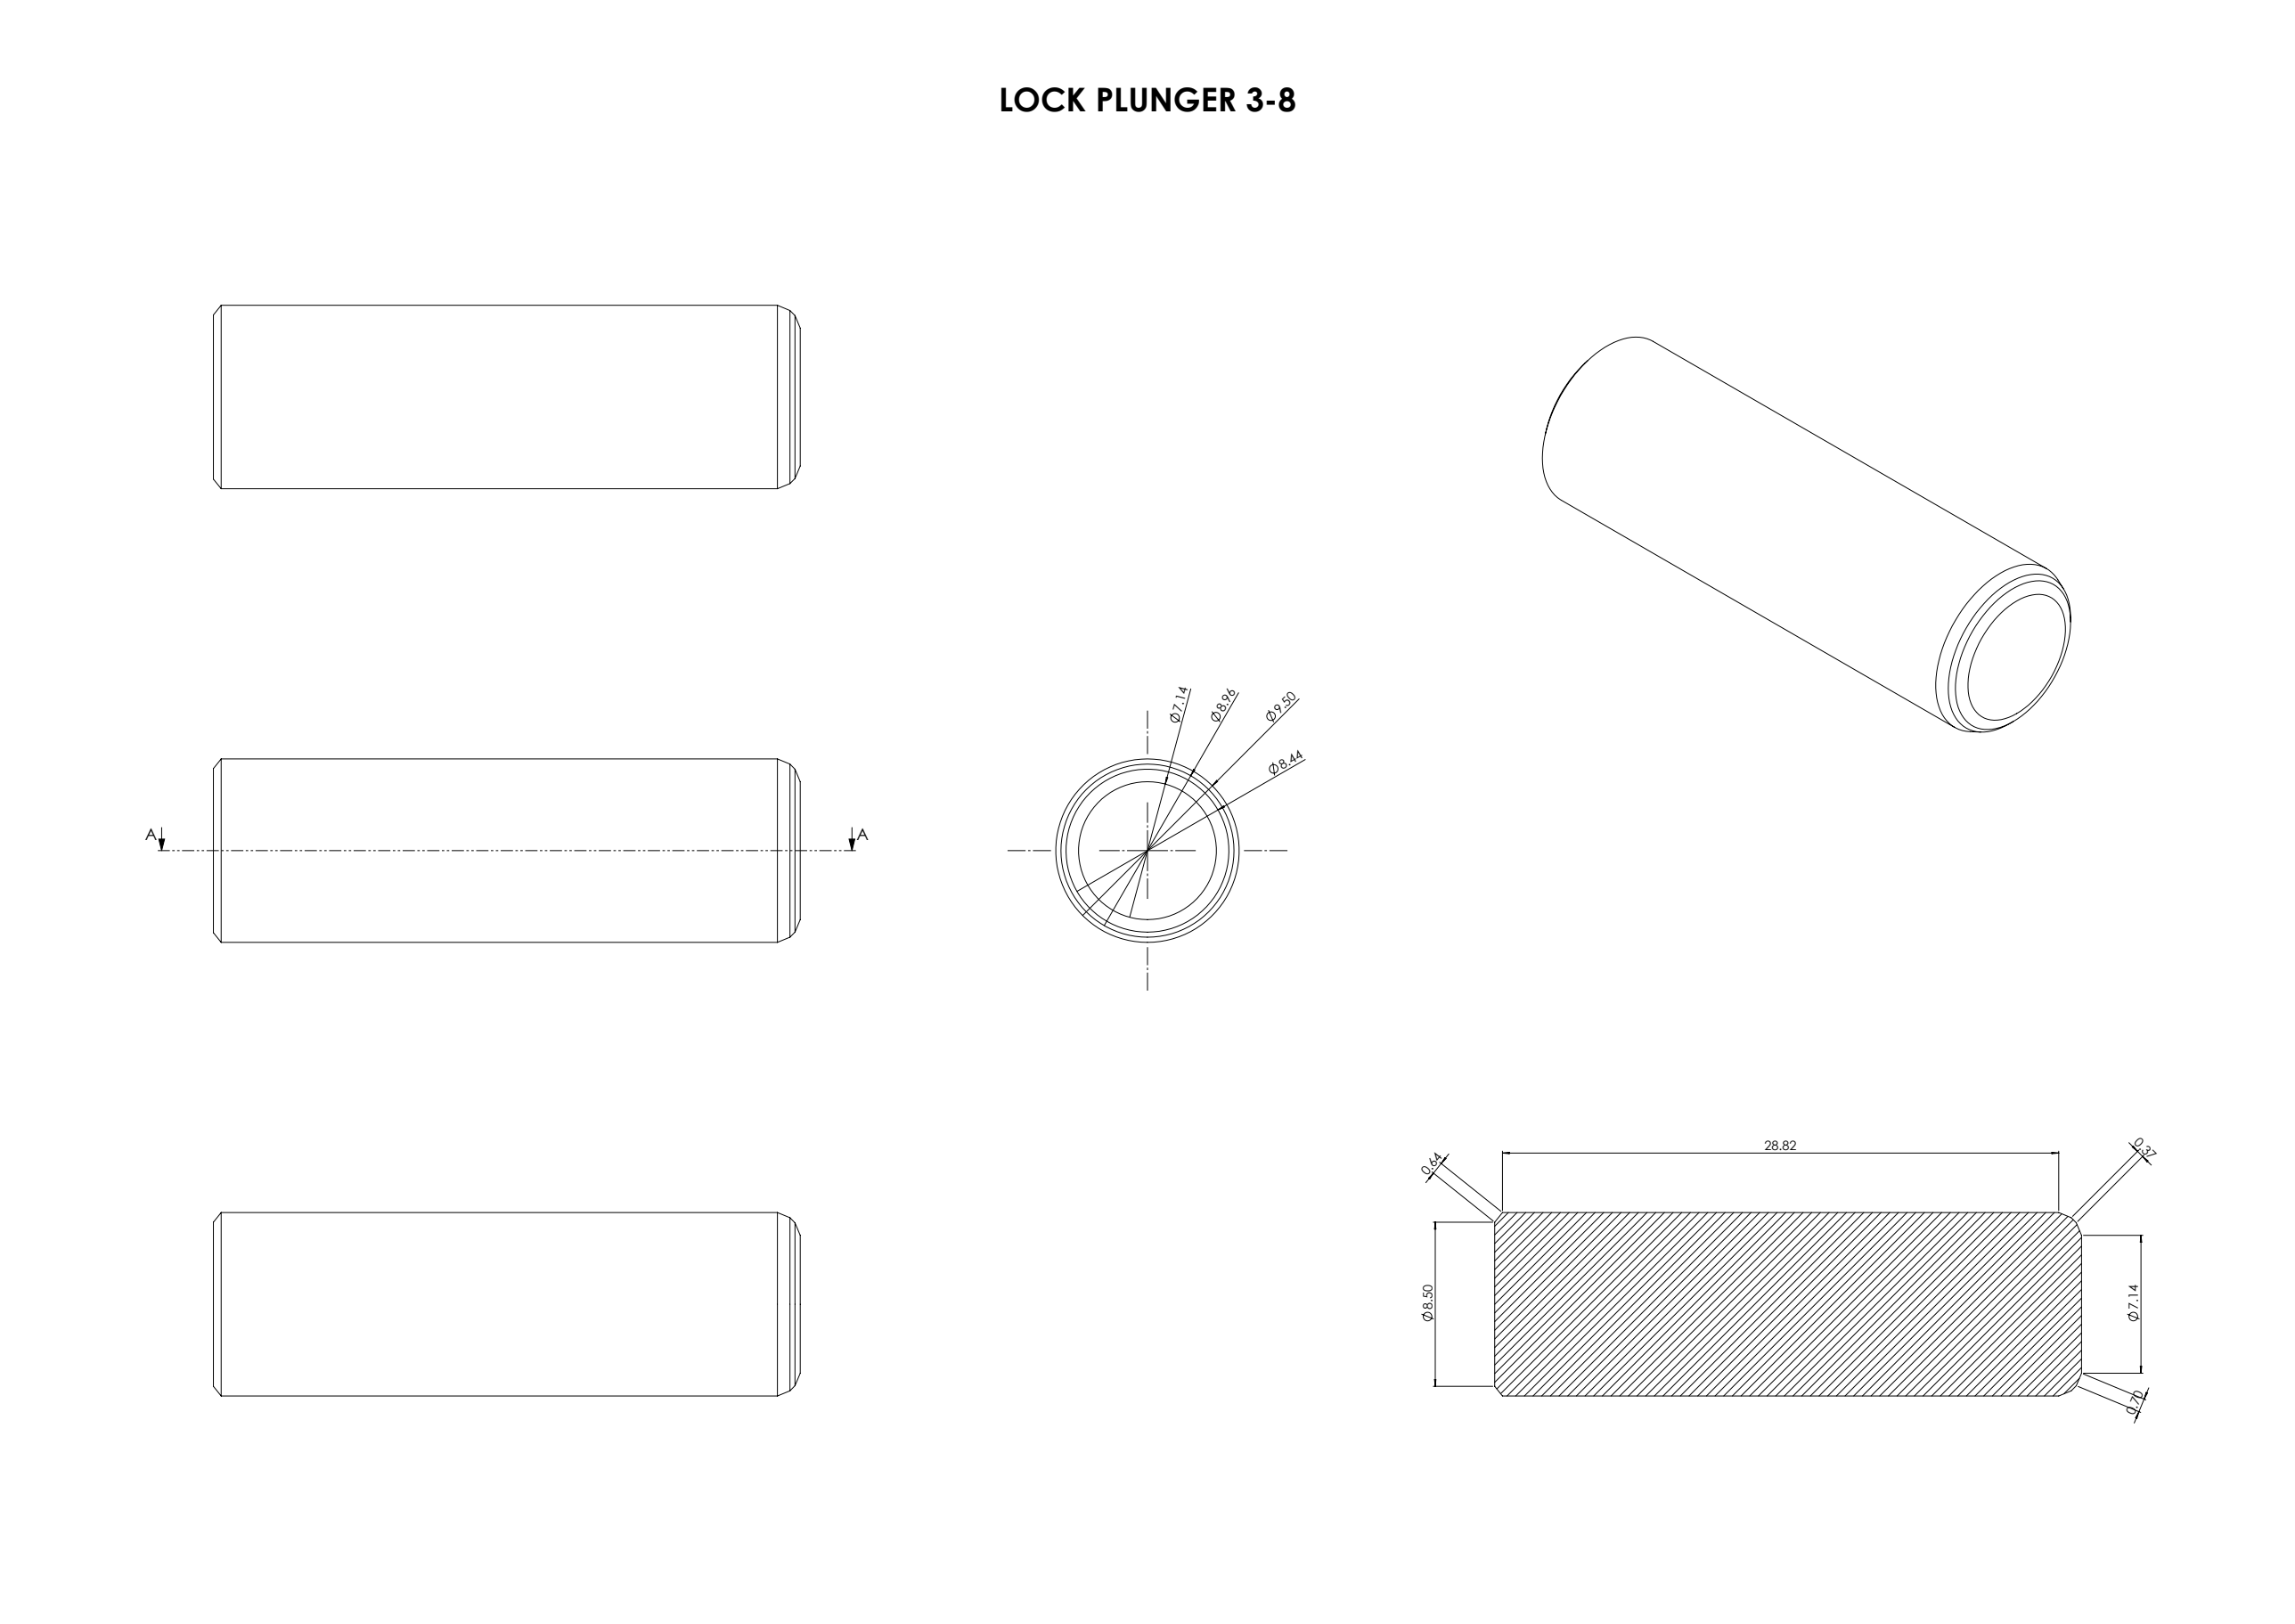
ISO-10303-21;
HEADER;
/* Generated by software containing ST-Developer
 * from STEP Tools, Inc. (www.steptools.com) 
 */

FILE_DESCRIPTION(
/* description */ (''),
/* implementation_level */ '2;1');

FILE_NAME(
/* name */ '09_Lock_Plunger_3-8.step',
/* time_stamp */ '2026-10-25T01:30:15-07:00',
/* author */ (''),
/* organization */ (''),
/* preprocessor_version */ 'ST-DEVELOPER v20.2',
/* originating_system */ 'Autodesk Translation Framework v15.15.0.0',
/* authorisation */ '');

FILE_SCHEMA (('AUTOMOTIVE_DESIGN { 1 0 10303 214 3 1 1 }'));
ENDSEC;

DATA;
#10=MECHANICAL_DESIGN_GEOMETRIC_PRESENTATION_REPRESENTATION('',(#571),#32309);
#543=SHAPE_REPRESENTATION_RELATIONSHIP('SRR','None',#32370,#557);
#557=ADVANCED_BREP_SHAPE_REPRESENTATION('',(#585),#32303);
#571=STYLED_ITEM('',(#32495),#585);
#585=MANIFOLD_SOLID_BREP('Body1',#13812);
#742=CYLINDRICAL_SURFACE('',#14622,4.75);
#1008=CIRCLE('',#14612,3.57);
#1009=CIRCLE('',#14613,4.21870057685089);
#1010=CIRCLE('',#14614,4.21870057685089);
#1011=CIRCLE('',#14616,4.48129942314911);
#1012=CIRCLE('',#14617,4.48129942314911);
#1013=CIRCLE('',#14620,4.75);
#1014=CIRCLE('',#14621,4.75);
#1015=CIRCLE('',#14623,4.75);
#1016=CIRCLE('',#14625,4.25);
#1202=CONICAL_SURFACE('',#14611,3.89435028842544,1.17809724509617);
#1203=CONICAL_SURFACE('',#14615,4.35,0.785398163397448);
#1204=CONICAL_SURFACE('',#14619,4.61564971157455,0.39269908169873);
#1205=CONICAL_SURFACE('',#14626,4.5,0.896055384571344);
#1711=FACE_OUTER_BOUND('',#2561,.T.);
#1712=FACE_OUTER_BOUND('',#2562,.T.);
#1713=FACE_OUTER_BOUND('',#2563,.T.);
#1714=FACE_OUTER_BOUND('',#2564,.T.);
#1715=FACE_OUTER_BOUND('',#2565,.T.);
#1716=FACE_OUTER_BOUND('',#2566,.T.);
#1717=FACE_OUTER_BOUND('',#2567,.T.);
#2561=EDGE_LOOP('',(#10909,#10910,#10911,#10912,#10913));
#2562=EDGE_LOOP('',(#10914,#10915,#10916,#10917,#10918,#10919));
#2563=EDGE_LOOP('',(#10920));
#2564=EDGE_LOOP('',(#10921,#10922,#10923,#10924,#10925,#10926));
#2565=EDGE_LOOP('',(#10927,#10928,#10929,#10930,#10931));
#2566=EDGE_LOOP('',(#10932));
#2567=EDGE_LOOP('',(#10933,#10934,#10935,#10936));
#3560=LINE('',#26498,#4871);
#3561=LINE('',#26504,#4872);
#3562=LINE('',#26511,#4873);
#3563=LINE('',#26517,#4874);
#3564=LINE('',#26523,#4875);
#4871=VECTOR('',#16948,3.89435028842544);
#4872=VECTOR('',#16955,4.35);
#4873=VECTOR('',#16964,4.61564971157455);
#4874=VECTOR('',#16971,4.75);
#4875=VECTOR('',#16980,4.5);
#6185=VERTEX_POINT('',#26495);
#6186=VERTEX_POINT('',#26497);
#6187=VERTEX_POINT('',#26499);
#6188=VERTEX_POINT('',#26503);
#6189=VERTEX_POINT('',#26505);
#6190=VERTEX_POINT('',#26510);
#6191=VERTEX_POINT('',#26512);
#6192=VERTEX_POINT('',#26516);
#6193=VERTEX_POINT('',#26520);
#7831=EDGE_CURVE('',#6185,#6185,#1008,.T.);
#7832=EDGE_CURVE('',#6185,#6186,#3560,.T.);
#7833=EDGE_CURVE('',#6186,#6187,#1009,.T.);
#7834=EDGE_CURVE('',#6187,#6186,#1010,.T.);
#7835=EDGE_CURVE('',#6187,#6188,#3561,.T.);
#7836=EDGE_CURVE('',#6189,#6188,#1011,.T.);
#7837=EDGE_CURVE('',#6188,#6189,#1012,.T.);
#7838=EDGE_CURVE('',#6189,#6190,#3562,.T.);
#7839=EDGE_CURVE('',#6190,#6191,#1013,.T.);
#7840=EDGE_CURVE('',#6191,#6190,#1014,.T.);
#7841=EDGE_CURVE('',#6191,#6192,#3563,.T.);
#7842=EDGE_CURVE('',#6192,#6192,#1015,.T.);
#7843=EDGE_CURVE('',#6193,#6193,#1016,.T.);
#7844=EDGE_CURVE('',#6192,#6193,#3564,.T.);
#10909=ORIENTED_EDGE('',*,*,#7831,.T.);
#10910=ORIENTED_EDGE('',*,*,#7832,.T.);
#10911=ORIENTED_EDGE('',*,*,#7833,.T.);
#10912=ORIENTED_EDGE('',*,*,#7834,.T.);
#10913=ORIENTED_EDGE('',*,*,#7832,.F.);
#10914=ORIENTED_EDGE('',*,*,#7833,.F.);
#10915=ORIENTED_EDGE('',*,*,#7834,.F.);
#10916=ORIENTED_EDGE('',*,*,#7835,.T.);
#10917=ORIENTED_EDGE('',*,*,#7836,.F.);
#10918=ORIENTED_EDGE('',*,*,#7837,.F.);
#10919=ORIENTED_EDGE('',*,*,#7835,.F.);
#10920=ORIENTED_EDGE('',*,*,#7831,.F.);
#10921=ORIENTED_EDGE('',*,*,#7836,.T.);
#10922=ORIENTED_EDGE('',*,*,#7837,.T.);
#10923=ORIENTED_EDGE('',*,*,#7838,.T.);
#10924=ORIENTED_EDGE('',*,*,#7839,.T.);
#10925=ORIENTED_EDGE('',*,*,#7840,.T.);
#10926=ORIENTED_EDGE('',*,*,#7838,.F.);
#10927=ORIENTED_EDGE('',*,*,#7839,.F.);
#10928=ORIENTED_EDGE('',*,*,#7840,.F.);
#10929=ORIENTED_EDGE('',*,*,#7841,.T.);
#10930=ORIENTED_EDGE('',*,*,#7842,.T.);
#10931=ORIENTED_EDGE('',*,*,#7841,.F.);
#10932=ORIENTED_EDGE('',*,*,#7843,.F.);
#10933=ORIENTED_EDGE('',*,*,#7842,.F.);
#10934=ORIENTED_EDGE('',*,*,#7844,.T.);
#10935=ORIENTED_EDGE('',*,*,#7843,.T.);
#10936=ORIENTED_EDGE('',*,*,#7844,.F.);
#12794=PLANE('',#14618);
#12795=PLANE('',#14624);
#13474=ADVANCED_FACE('',(#1711),#1202,.T.);
#13475=ADVANCED_FACE('',(#1712),#1203,.T.);
#13476=ADVANCED_FACE('',(#1713),#12794,.T.);
#13477=ADVANCED_FACE('',(#1714),#1204,.T.);
#13478=ADVANCED_FACE('',(#1715),#742,.T.);
#13479=ADVANCED_FACE('',(#1716),#12795,.T.);
#13480=ADVANCED_FACE('',(#1717),#1205,.T.);
#13812=CLOSED_SHELL('',(#13474,#13475,#13476,#13477,#13478,#13479,#13480));
#14610=AXIS2_PLACEMENT_3D('',#26493,#16942,#16943);
#14611=AXIS2_PLACEMENT_3D('',#26494,#16944,#16945);
#14612=AXIS2_PLACEMENT_3D('',#26496,#16946,#16947);
#14613=AXIS2_PLACEMENT_3D('',#26500,#16949,#16950);
#14614=AXIS2_PLACEMENT_3D('',#26501,#16951,#16952);
#14615=AXIS2_PLACEMENT_3D('',#26502,#16953,#16954);
#14616=AXIS2_PLACEMENT_3D('',#26506,#16956,#16957);
#14617=AXIS2_PLACEMENT_3D('',#26507,#16958,#16959);
#14618=AXIS2_PLACEMENT_3D('',#26508,#16960,#16961);
#14619=AXIS2_PLACEMENT_3D('',#26509,#16962,#16963);
#14620=AXIS2_PLACEMENT_3D('',#26513,#16965,#16966);
#14621=AXIS2_PLACEMENT_3D('',#26514,#16967,#16968);
#14622=AXIS2_PLACEMENT_3D('',#26515,#16969,#16970);
#14623=AXIS2_PLACEMENT_3D('',#26518,#16972,#16973);
#14624=AXIS2_PLACEMENT_3D('',#26519,#16974,#16975);
#14625=AXIS2_PLACEMENT_3D('',#26521,#16976,#16977);
#14626=AXIS2_PLACEMENT_3D('',#26522,#16978,#16979);
#16942=DIRECTION('axis',(0.,0.,1.));
#16943=DIRECTION('refdir',(1.,0.,0.));
#16944=DIRECTION('center_axis',(-1.,0.,-9.61370872096891E-16));
#16945=DIRECTION('ref_axis',(0.,-1.,-3.31661110028857E-17));
#16946=DIRECTION('center_axis',(-1.,0.,0.));
#16947=DIRECTION('ref_axis',(0.,-1.,0.));
#16948=DIRECTION('',(-0.38268343236509,0.923879532511287,-2.24116602752525E-16));
#16949=DIRECTION('center_axis',(1.,0.,0.));
#16950=DIRECTION('ref_axis',(0.,-1.,-6.12323399573677E-17));
#16951=DIRECTION('center_axis',(1.,0.,0.));
#16952=DIRECTION('ref_axis',(0.,-1.,-6.12323399573677E-17));
#16953=DIRECTION('center_axis',(-1.,0.,0.));
#16954=DIRECTION('ref_axis',(0.,1.,0.));
#16955=DIRECTION('',(-0.707106781186548,-0.707106781186547,-8.65956056235493E-17));
#16956=DIRECTION('center_axis',(-1.,0.,0.));
#16957=DIRECTION('ref_axis',(0.,-1.,-6.12323399573677E-17));
#16958=DIRECTION('center_axis',(-1.,0.,0.));
#16959=DIRECTION('ref_axis',(0.,-1.,-6.12323399573677E-17));
#16960=DIRECTION('center_axis',(1.,0.,0.));
#16961=DIRECTION('ref_axis',(0.,0.,-1.));
#16962=DIRECTION('center_axis',(-1.,0.,4.23000162973647E-16));
#16963=DIRECTION('ref_axis',(0.,-1.,-2.9725008056928E-17));
#16964=DIRECTION('',(-0.923879532511284,0.382683432365095,4.49041664983859E-16));
#16965=DIRECTION('center_axis',(1.,0.,0.));
#16966=DIRECTION('ref_axis',(0.,-1.,0.));
#16967=DIRECTION('center_axis',(1.,0.,0.));
#16968=DIRECTION('ref_axis',(0.,-1.,0.));
#16969=DIRECTION('center_axis',(1.,0.,0.));
#16970=DIRECTION('ref_axis',(0.,1.,0.));
#16971=DIRECTION('',(-1.,0.,0.));
#16972=DIRECTION('center_axis',(1.,0.,0.));
#16973=DIRECTION('ref_axis',(0.,0.,-1.));
#16974=DIRECTION('center_axis',(-1.,0.,0.));
#16975=DIRECTION('ref_axis',(0.,0.,1.));
#16976=DIRECTION('center_axis',(1.,0.,0.));
#16977=DIRECTION('ref_axis',(0.,0.,-1.));
#16978=DIRECTION('center_axis',(1.,0.,0.));
#16979=DIRECTION('ref_axis',(0.,1.,0.));
#16980=DIRECTION('',(-0.624695047554424,0.78086880944303,9.56288488038411E-17));
#26493=CARTESIAN_POINT('',(0.,0.,0.));
#26494=CARTESIAN_POINT('Origin',(30.2656497115746,0.,-1.29160453950038E-16));
#26495=CARTESIAN_POINT('',(30.4,3.57,-4.37198907295605E-16));
#26496=CARTESIAN_POINT('Origin',(30.4,0.,0.));
#26497=CARTESIAN_POINT('',(30.1312994231491,4.21870057685089,5.16641815800153E-16));
#26498=CARTESIAN_POINT('',(30.2656497115746,3.89435028842544,4.76920361547879E-16));
#26499=CARTESIAN_POINT('',(30.1312994231491,-4.21870057685089,-5.16641815800153E-16));
#26500=CARTESIAN_POINT('Origin',(30.1312994231491,0.,-2.58320907900077E-16));
#26501=CARTESIAN_POINT('Origin',(30.1312994231491,0.,-2.58320907900077E-16));
#26502=CARTESIAN_POINT('Origin',(30.,0.,0.));
#26503=CARTESIAN_POINT('',(29.8687005768509,-4.48129942314911,-5.48800899458044E-16));
#26504=CARTESIAN_POINT('',(30.,-4.35,-5.32721357629099E-16));
#26505=CARTESIAN_POINT('',(29.8687005768509,4.48129942314911,-5.48800899458044E-16));
#26506=CARTESIAN_POINT('Origin',(29.8687005768509,0.,-2.74400449729022E-16));
#26507=CARTESIAN_POINT('Origin',(29.8687005768509,0.,-2.74400449729022E-16));
#26508=CARTESIAN_POINT('Origin',(30.4,0.,0.));
#26509=CARTESIAN_POINT('Origin',(29.5443502884254,0.,-1.37200224864511E-16));
#26510=CARTESIAN_POINT('',(29.22,4.75,5.81707229594993E-16));
#26511=CARTESIAN_POINT('',(29.5443502884254,4.61564971157455,5.65254064526518E-16));
#26512=CARTESIAN_POINT('',(29.22,-4.75,-5.81707229594993E-16));
#26513=CARTESIAN_POINT('Origin',(29.22,0.,0.));
#26514=CARTESIAN_POINT('Origin',(29.22,0.,0.));
#26515=CARTESIAN_POINT('Origin',(15.,0.,0.));
#26516=CARTESIAN_POINT('',(0.4,-4.75,-5.81707229594993E-16));
#26517=CARTESIAN_POINT('',(15.,-4.75,-5.81707229594993E-16));
#26518=CARTESIAN_POINT('Origin',(0.4,0.,0.));
#26519=CARTESIAN_POINT('Origin',(0.,4.25,0.));
#26520=CARTESIAN_POINT('',(1.04083408558608E-16,-4.25,-5.20474889637625E-16));
#26521=CARTESIAN_POINT('Origin',(0.,0.,0.));
#26522=CARTESIAN_POINT('Origin',(0.2,0.,0.));
#26523=CARTESIAN_POINT('',(0.2,-4.5,-5.51091059616309E-16));
#32287=UNCERTAINTY_MEASURE_WITH_UNIT(LENGTH_MEASURE(0.01),#32310,
'DISTANCE_ACCURACY_VALUE',
'Maximum model space distance between geometric entities at asserted c
onnectivities');
#32293=UNCERTAINTY_MEASURE_WITH_UNIT(LENGTH_MEASURE(0.01),#32310,
'DISTANCE_ACCURACY_VALUE',
'Maximum model space distance between geometric entities at asserted c
onnectivities');
#32303=(
GEOMETRIC_REPRESENTATION_CONTEXT(3)
GLOBAL_UNCERTAINTY_ASSIGNED_CONTEXT((#32287))
GLOBAL_UNIT_ASSIGNED_CONTEXT((#32310,#32312,#32313))
REPRESENTATION_CONTEXT('','3D')
);
#32309=(
GEOMETRIC_REPRESENTATION_CONTEXT(3)
GLOBAL_UNCERTAINTY_ASSIGNED_CONTEXT((#32293))
GLOBAL_UNIT_ASSIGNED_CONTEXT((#32310,#32312,#32313))
REPRESENTATION_CONTEXT('','3D')
);
#32310=(
LENGTH_UNIT()
NAMED_UNIT(*)
SI_UNIT(.MILLI.,.METRE.)
);
#32312=(
NAMED_UNIT(*)
PLANE_ANGLE_UNIT()
SI_UNIT($,.RADIAN.)
);
#32313=(
NAMED_UNIT(*)
SI_UNIT($,.STERADIAN.)
SOLID_ANGLE_UNIT()
);
#32323=SHAPE_DEFINITION_REPRESENTATION(#32338,#32370);
#32338=PRODUCT_DEFINITION_SHAPE('',$,#32386);
#32370=SHAPE_REPRESENTATION('',(#14610),#32303);
#32376=PRODUCT_DEFINITION_CONTEXT('part definition',#32423,'design');
#32386=PRODUCT_DEFINITION('2026-10-25-00-35-19-682',
'09_Lock_Plunger_3-8',#32401,#32376);
#32401=PRODUCT_DEFINITION_FORMATION('',$,#32434);
#32423=APPLICATION_CONTEXT(
'Core Data for Automotive Mechanical Design Process');
#32424=PRODUCT_CONTEXT('part definition',#32423,'mechanical');
#32434=PRODUCT('2026-10-25-00-35-19-682','09_Lock_Plunger_3-8',$,(#32424));
#32489=COLOUR_RGB('Sky Blue',0.24,0.69,0.87);
#32490=FILL_AREA_STYLE_COLOUR('',#32489);
#32491=FILL_AREA_STYLE('',(#32490));
#32492=SURFACE_STYLE_FILL_AREA(#32491);
#32493=SURFACE_SIDE_STYLE('',(#32492));
#32494=SURFACE_STYLE_USAGE(.BOTH.,#32493);
#32495=PRESENTATION_STYLE_ASSIGNMENT((#32494));
ENDSEC;
END-ISO-10303-21;
